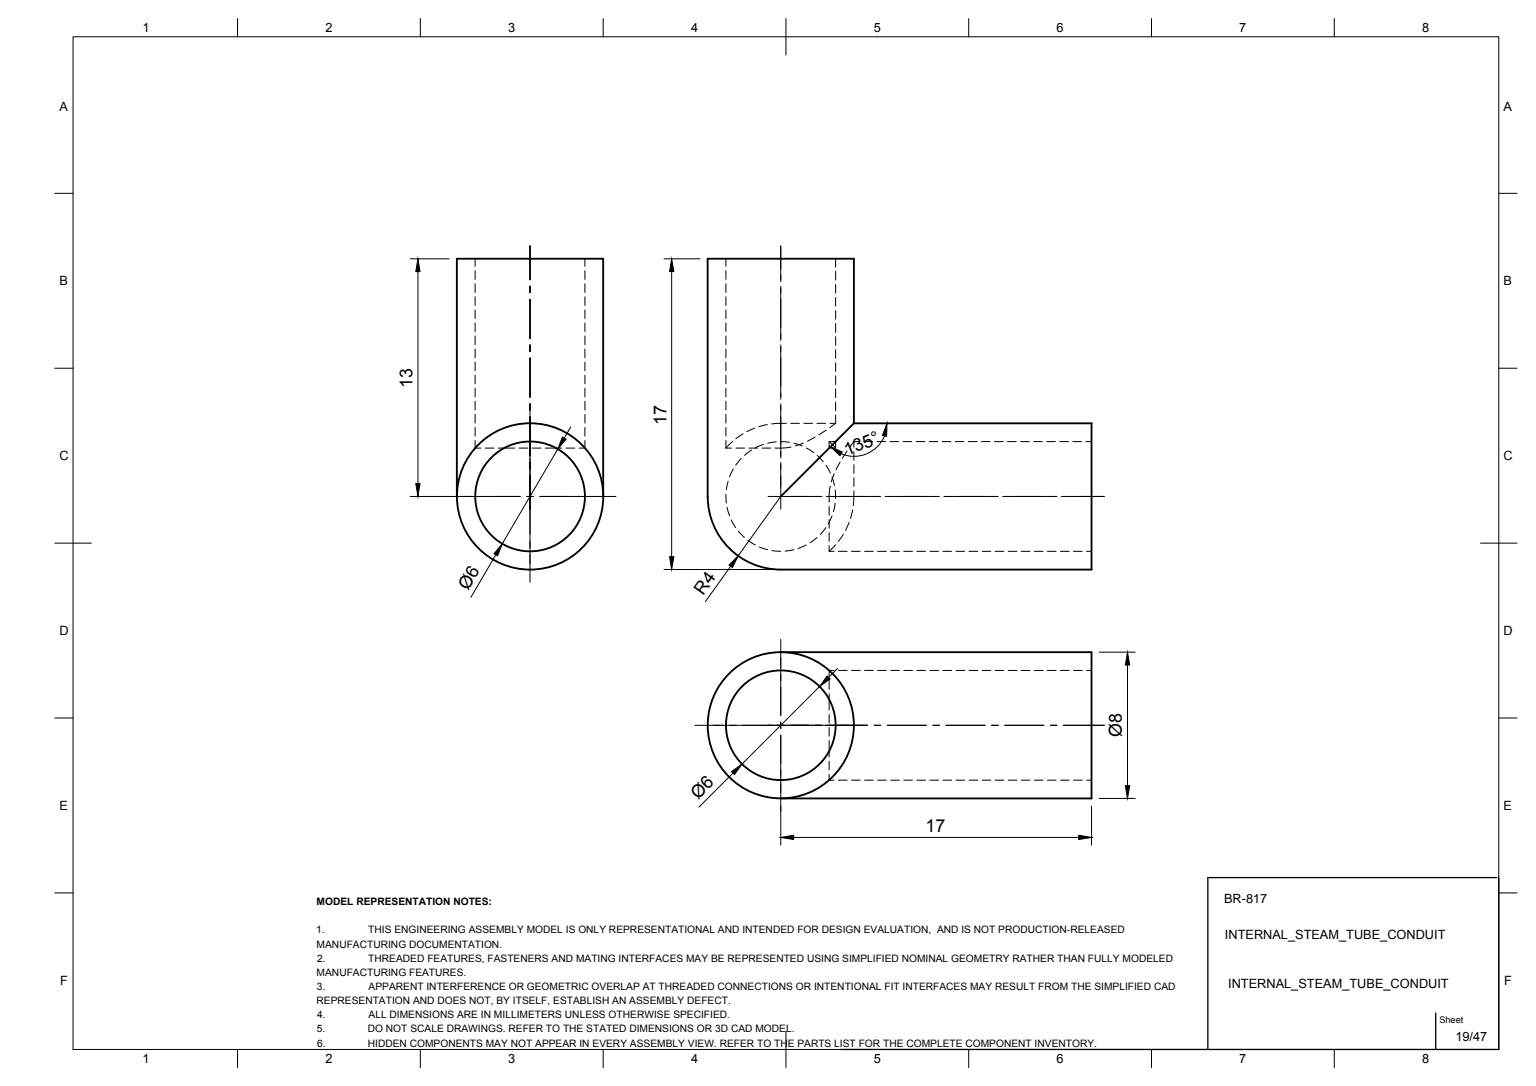
ISO-10303-21;
HEADER;
FILE_DESCRIPTION((''),'2;1');
FILE_NAME('INTERNAL_STEAM_TUBE_CONDUIT.step','2026-10-01T22:07:29-07:00',(''),(''),'','','');
FILE_SCHEMA (('AUTOMOTIVE_DESIGN { 1 0 10303 214 3 1 1 }'));
ENDSEC;
DATA;
#10=MECHANICAL_DESIGN_GEOMETRIC_PRESENTATION_REPRESENTATION('',(#553),#15484);
#11=B_SPLINE_CURVE_WITH_KNOTS('',3,(#13547,#13548,#13549,#13550,#13551,
#13552,#13553,#13554,#13555,#13556,#13557,#13558,#13559,#13560,#13561,#13562,
#13563,#13564,#13565,#13566,#13567,#13568),.UNSPECIFIED.,.F.,.F.,(4,2,2,
2,2,2,2,2,2,2,4),(-0.956775615070491,-0.896341583425282,-0.835907551780074,
-0.715039488489657,-0.596713648012451,-0.478387807535245,-0.36006196705804,
-0.241736126580834,-0.120868063290417,-0.0604340316452086,0.),
 .UNSPECIFIED.) ;
#12=B_SPLINE_CURVE_WITH_KNOTS('',3,(#13586,#13587,#13588,#13589,#13590,
#13591,#13592,#13593,#13594,#13595,#13596,#13597,#13598,#13599,#13600,#13601,
#13602,#13603,#13604,#13605,#13606,#13607),.UNSPECIFIED.,.F.,.F.,(4,2,2,
2,2,2,2,2,2,2,4),(0.,0.0604340316452085,0.120868063290417,0.241736126580834,
0.36006196705804,0.478387807535245,0.596713648012451,0.715039488489657,
0.835907551780074,0.896341583425282,0.956775615070491),.UNSPECIFIED.) ;
#13=ELLIPSE('',#8939,0.424264068711929,0.3) ;
#14=ELLIPSE('',#8947,0.565685424949238,0.4) ;
#189=ORIENTED_CLOSED_SHELL('',*,#8262,.F.) ;
#190=ORIENTED_CLOSED_SHELL('',*,#8263,.F.) ;
#191=BREP_WITH_VOIDS('INTERNAL_STEAM_TUBE_CONDUIT',#8264,(#189,#190)) ;
#193=SPHERICAL_SURFACE('',#8933,0.3) ;
#194=SPHERICAL_SURFACE('',#8935,0.4) ;
#195=SPHERICAL_SURFACE('',#8964,0.4) ;
#196=SPHERICAL_SURFACE('',#8965,0.4) ;
#197=SPHERICAL_SURFACE('',#8966,0.4) ;
#483=SHAPE_REPRESENTATION_RELATIONSHIP('SRR','None',#15632,#518) ;
#518=ADVANCED_BREP_SHAPE_REPRESENTATION('',(#191),#15456) ;
#553=STYLED_ITEM('',(#15836),#191) ;
#667=CYLINDRICAL_SURFACE('',#8938,0.3) ;
#668=CYLINDRICAL_SURFACE('',#8940,0.3) ;
#669=CYLINDRICAL_SURFACE('',#8944,0.4) ;
#670=CYLINDRICAL_SURFACE('',#8946,0.4) ;
#671=CYLINDRICAL_SURFACE('',#8953,0.4) ;
#672=CYLINDRICAL_SURFACE('',#8955,0.4) ;
#673=CYLINDRICAL_SURFACE('',#8958,0.3) ;
#674=CYLINDRICAL_SURFACE('',#8961,0.3) ;
#859=FACE_BOUND('',#2058,.T.) ;
#860=FACE_BOUND('',#2062,.T.) ;
#976=CIRCLE('',#8934,0.3) ;
#977=CIRCLE('',#8936,0.3) ;
#978=CIRCLE('',#8937,0.3) ;
#979=CIRCLE('',#8942,0.4) ;
#980=CIRCLE('',#8943,0.3) ;
#981=CIRCLE('',#8945,0.4) ;
#982=CIRCLE('',#8948,0.4) ;
#983=CIRCLE('',#8949,0.4) ;
#984=CIRCLE('',#8951,0.4) ;
#985=CIRCLE('',#8952,0.3) ;
#986=CIRCLE('',#8954,0.4) ;
#987=CIRCLE('',#8956,0.4) ;
#988=CIRCLE('',#8957,0.4) ;
#989=CIRCLE('',#8959,0.3) ;
#990=CIRCLE('',#8960,0.3) ;
#991=CIRCLE('',#8962,0.3) ;
#992=CIRCLE('',#8963,0.3) ;
#1504=FACE_OUTER_BOUND('',#2053,.T.) ;
#1505=FACE_OUTER_BOUND('',#2054,.T.) ;
#1506=FACE_OUTER_BOUND('',#2055,.T.) ;
#1507=FACE_OUTER_BOUND('',#2056,.T.) ;
#1508=FACE_OUTER_BOUND('',#2057,.T.) ;
#1509=FACE_OUTER_BOUND('',#2059,.T.) ;
#1510=FACE_OUTER_BOUND('',#2060,.T.) ;
#1511=FACE_OUTER_BOUND('',#2061,.T.) ;
#1512=FACE_OUTER_BOUND('',#2063,.T.) ;
#1513=FACE_OUTER_BOUND('',#2064,.T.) ;
#1514=FACE_OUTER_BOUND('',#2065,.T.) ;
#1515=FACE_OUTER_BOUND('',#2066,.T.) ;
#1516=FACE_OUTER_BOUND('',#2067,.T.) ;
#1517=FACE_OUTER_BOUND('',#2068,.T.) ;
#1518=FACE_OUTER_BOUND('',#2069,.T.) ;
#2053=EDGE_LOOP('',(#5851,#5852)) ;
#2054=EDGE_LOOP('',(#5853,#5854)) ;
#2055=EDGE_LOOP('',(#5855,#5856)) ;
#2056=EDGE_LOOP('',(#5857,#5858)) ;
#2057=EDGE_LOOP('',(#5859)) ;
#2058=EDGE_LOOP('',(#5860)) ;
#2059=EDGE_LOOP('',(#5861,#5862)) ;
#2060=EDGE_LOOP('',(#5863,#5864,#5865,#5866,#5867,#5868)) ;
#2061=EDGE_LOOP('',(#5869)) ;
#2062=EDGE_LOOP('',(#5870)) ;
#2063=EDGE_LOOP('',(#5871,#5872)) ;
#2064=EDGE_LOOP('',(#5873,#5874,#5875,#5876,#5877,#5878)) ;
#2065=EDGE_LOOP('',(#5879,#5880,#5881,#5882,#5883,#5884)) ;
#2066=EDGE_LOOP('',(#5885,#5886,#5887,#5888,#5889,#5890)) ;
#2067=EDGE_LOOP('',(#5891,#5892,#5893,#5894)) ;
#2068=EDGE_LOOP('',(#5895,#5896,#5897)) ;
#2069=EDGE_LOOP('',(#5898,#5899,#5900)) ;
#2638=LINE('',#13576,#3112) ;
#2639=LINE('',#13611,#3113) ;
#2640=LINE('',#13617,#3114) ;
#2641=LINE('',#13621,#3115) ;
#3112=VECTOR('',#10657,0.4) ;
#3113=VECTOR('',#10672,0.4) ;
#3114=VECTOR('',#10681,0.3) ;
#3115=VECTOR('',#10686,0.3) ;
#3581=VERTEX_POINT('',#13528) ;
#3582=VERTEX_POINT('',#13529) ;
#3583=VERTEX_POINT('',#13532) ;
#3584=VERTEX_POINT('',#13533) ;
#3585=VERTEX_POINT('',#13540) ;
#3586=VERTEX_POINT('',#13542) ;
#3587=VERTEX_POINT('',#13545) ;
#3588=VERTEX_POINT('',#13546) ;
#3589=VERTEX_POINT('',#13571) ;
#3590=VERTEX_POINT('',#13572) ;
#3591=VERTEX_POINT('',#13574) ;
#3592=VERTEX_POINT('',#13579) ;
#3593=VERTEX_POINT('',#13581) ;
#3594=VERTEX_POINT('',#13584) ;
#3595=VERTEX_POINT('',#13585) ;
#3596=VERTEX_POINT('',#13610) ;
#3597=VERTEX_POINT('',#13615) ;
#3598=VERTEX_POINT('',#13620) ;
#4430=EDGE_CURVE('',#3581,#3582,#976,.T.) ;
#4431=EDGE_CURVE('',#3583,#3584,#977,.T.) ;
#4432=EDGE_CURVE('',#3584,#3583,#978,.T.) ;
#4433=EDGE_CURVE('',#3583,#3584,#13,.T.) ;
#4434=EDGE_CURVE('',#3585,#3585,#979,.T.) ;
#4435=EDGE_CURVE('',#3586,#3586,#980,.T.) ;
#4436=EDGE_CURVE('',#3587,#3588,#11,.T.) ;
#4437=EDGE_CURVE('',#3587,#3588,#981,.T.) ;
#4438=EDGE_CURVE('',#3589,#3590,#14,.T.) ;
#4439=EDGE_CURVE('',#3591,#3590,#982,.T.) ;
#4440=EDGE_CURVE('',#3591,#3585,#2638,.T.) ;
#4441=EDGE_CURVE('',#3589,#3591,#983,.T.) ;
#4442=EDGE_CURVE('',#3592,#3592,#984,.T.) ;
#4443=EDGE_CURVE('',#3593,#3593,#985,.T.) ;
#4444=EDGE_CURVE('',#3594,#3595,#12,.T.) ;
#4445=EDGE_CURVE('',#3595,#3594,#986,.T.) ;
#4446=EDGE_CURVE('',#3592,#3596,#2639,.T.) ;
#4447=EDGE_CURVE('',#3590,#3596,#987,.T.) ;
#4448=EDGE_CURVE('',#3596,#3589,#988,.T.) ;
#4449=EDGE_CURVE('',#3587,#3597,#989,.T.) ;
#4450=EDGE_CURVE('',#3597,#3593,#2640,.T.) ;
#4451=EDGE_CURVE('',#3597,#3588,#990,.T.) ;
#4452=EDGE_CURVE('',#3586,#3598,#2641,.T.) ;
#4453=EDGE_CURVE('',#3598,#3594,#991,.T.) ;
#4454=EDGE_CURVE('',#3595,#3598,#992,.T.) ;
#5851=ORIENTED_EDGE('',*,*,#4430,.T.) ;
#5852=ORIENTED_EDGE('',*,*,#4430,.F.) ;
#5853=ORIENTED_EDGE('',*,*,#4431,.F.) ;
#5854=ORIENTED_EDGE('',*,*,#4432,.F.) ;
#5855=ORIENTED_EDGE('',*,*,#4432,.T.) ;
#5856=ORIENTED_EDGE('',*,*,#4433,.T.) ;
#5857=ORIENTED_EDGE('',*,*,#4431,.T.) ;
#5858=ORIENTED_EDGE('',*,*,#4433,.F.) ;
#5859=ORIENTED_EDGE('',*,*,#4434,.T.) ;
#5860=ORIENTED_EDGE('',*,*,#4435,.T.) ;
#5861=ORIENTED_EDGE('',*,*,#4436,.T.) ;
#5862=ORIENTED_EDGE('',*,*,#4437,.F.) ;
#5863=ORIENTED_EDGE('',*,*,#4438,.T.) ;
#5864=ORIENTED_EDGE('',*,*,#4439,.F.) ;
#5865=ORIENTED_EDGE('',*,*,#4440,.T.) ;
#5866=ORIENTED_EDGE('',*,*,#4434,.F.) ;
#5867=ORIENTED_EDGE('',*,*,#4440,.F.) ;
#5868=ORIENTED_EDGE('',*,*,#4441,.F.) ;
#5869=ORIENTED_EDGE('',*,*,#4442,.T.) ;
#5870=ORIENTED_EDGE('',*,*,#4443,.T.) ;
#5871=ORIENTED_EDGE('',*,*,#4444,.F.) ;
#5872=ORIENTED_EDGE('',*,*,#4445,.F.) ;
#5873=ORIENTED_EDGE('',*,*,#4442,.F.) ;
#5874=ORIENTED_EDGE('',*,*,#4446,.T.) ;
#5875=ORIENTED_EDGE('',*,*,#4447,.F.) ;
#5876=ORIENTED_EDGE('',*,*,#4438,.F.) ;
#5877=ORIENTED_EDGE('',*,*,#4448,.F.) ;
#5878=ORIENTED_EDGE('',*,*,#4446,.F.) ;
#5879=ORIENTED_EDGE('',*,*,#4449,.T.) ;
#5880=ORIENTED_EDGE('',*,*,#4450,.T.) ;
#5881=ORIENTED_EDGE('',*,*,#4443,.F.) ;
#5882=ORIENTED_EDGE('',*,*,#4450,.F.) ;
#5883=ORIENTED_EDGE('',*,*,#4451,.T.) ;
#5884=ORIENTED_EDGE('',*,*,#4436,.F.) ;
#5885=ORIENTED_EDGE('',*,*,#4435,.F.) ;
#5886=ORIENTED_EDGE('',*,*,#4452,.T.) ;
#5887=ORIENTED_EDGE('',*,*,#4453,.T.) ;
#5888=ORIENTED_EDGE('',*,*,#4444,.T.) ;
#5889=ORIENTED_EDGE('',*,*,#4454,.T.) ;
#5890=ORIENTED_EDGE('',*,*,#4452,.F.) ;
#5891=ORIENTED_EDGE('',*,*,#4447,.T.) ;
#5892=ORIENTED_EDGE('',*,*,#4448,.T.) ;
#5893=ORIENTED_EDGE('',*,*,#4441,.T.) ;
#5894=ORIENTED_EDGE('',*,*,#4439,.T.) ;
#5895=ORIENTED_EDGE('',*,*,#4449,.F.) ;
#5896=ORIENTED_EDGE('',*,*,#4437,.T.) ;
#5897=ORIENTED_EDGE('',*,*,#4451,.F.) ;
#5898=ORIENTED_EDGE('',*,*,#4445,.T.) ;
#5899=ORIENTED_EDGE('',*,*,#4453,.F.) ;
#5900=ORIENTED_EDGE('',*,*,#4454,.F.) ;
#7634=PLANE('',#8941) ;
#7635=PLANE('',#8950) ;
#7891=ADVANCED_FACE('',(#1504),#193,.F.) ;
#7892=ADVANCED_FACE('',(#1505),#194,.T.) ;
#7893=ADVANCED_FACE('',(#1506),#667,.F.) ;
#7894=ADVANCED_FACE('',(#1507),#668,.F.) ;
#7895=ADVANCED_FACE('',(#1508,#859),#7634,.T.) ;
#7896=ADVANCED_FACE('',(#1509),#669,.T.) ;
#7897=ADVANCED_FACE('',(#1510),#670,.T.) ;
#7898=ADVANCED_FACE('',(#1511,#860),#7635,.T.) ;
#7899=ADVANCED_FACE('',(#1512),#671,.T.) ;
#7900=ADVANCED_FACE('',(#1513),#672,.T.) ;
#7901=ADVANCED_FACE('',(#1514),#673,.F.) ;
#7902=ADVANCED_FACE('',(#1515),#674,.F.) ;
#7903=ADVANCED_FACE('',(#1516),#195,.T.) ;
#7904=ADVANCED_FACE('',(#1517),#196,.T.) ;
#7905=ADVANCED_FACE('',(#1518),#197,.T.) ;
#8262=CLOSED_SHELL('',(#7891)) ;
#8263=CLOSED_SHELL('',(#7892,#7893,#7894)) ;
#8264=CLOSED_SHELL('',(#7895,#7896,#7897,#7898,#7899,#7900,#7901,#7902,
#7903,#7904,#7905)) ;
#8932=AXIS2_PLACEMENT_3D('',#13526,#10623,#10624) ;
#8933=AXIS2_PLACEMENT_3D('',#13527,#10625,#10626) ;
#8934=AXIS2_PLACEMENT_3D('',#13530,#10627,#10628) ;
#8935=AXIS2_PLACEMENT_3D('',#13531,#10629,#10630) ;
#8936=AXIS2_PLACEMENT_3D('',#13534,#10631,#10632) ;
#8937=AXIS2_PLACEMENT_3D('',#13535,#10633,#10634) ;
#8938=AXIS2_PLACEMENT_3D('',#13536,#10635,#10636) ;
#8939=AXIS2_PLACEMENT_3D('',#13537,#10637,#10638) ;
#8940=AXIS2_PLACEMENT_3D('',#13538,#10639,#10640) ;
#8941=AXIS2_PLACEMENT_3D('',#13539,#10641,#10642) ;
#8942=AXIS2_PLACEMENT_3D('',#13541,#10643,#10644) ;
#8943=AXIS2_PLACEMENT_3D('',#13543,#10645,#10646) ;
#8944=AXIS2_PLACEMENT_3D('',#13544,#10647,#10648) ;
#8945=AXIS2_PLACEMENT_3D('',#13569,#10649,#10650) ;
#8946=AXIS2_PLACEMENT_3D('',#13570,#10651,#10652) ;
#8947=AXIS2_PLACEMENT_3D('',#13573,#10653,#10654) ;
#8948=AXIS2_PLACEMENT_3D('',#13575,#10655,#10656) ;
#8949=AXIS2_PLACEMENT_3D('',#13577,#10658,#10659) ;
#8950=AXIS2_PLACEMENT_3D('',#13578,#10660,#10661) ;
#8951=AXIS2_PLACEMENT_3D('',#13580,#10662,#10663) ;
#8952=AXIS2_PLACEMENT_3D('',#13582,#10664,#10665) ;
#8953=AXIS2_PLACEMENT_3D('',#13583,#10666,#10667) ;
#8954=AXIS2_PLACEMENT_3D('',#13608,#10668,#10669) ;
#8955=AXIS2_PLACEMENT_3D('',#13609,#10670,#10671) ;
#8956=AXIS2_PLACEMENT_3D('',#13612,#10673,#10674) ;
#8957=AXIS2_PLACEMENT_3D('',#13613,#10675,#10676) ;
#8958=AXIS2_PLACEMENT_3D('',#13614,#10677,#10678) ;
#8959=AXIS2_PLACEMENT_3D('',#13616,#10679,#10680) ;
#8960=AXIS2_PLACEMENT_3D('',#13618,#10682,#10683) ;
#8961=AXIS2_PLACEMENT_3D('',#13619,#10684,#10685) ;
#8962=AXIS2_PLACEMENT_3D('',#13622,#10687,#10688) ;
#8963=AXIS2_PLACEMENT_3D('',#13623,#10689,#10690) ;
#8964=AXIS2_PLACEMENT_3D('',#13624,#10691,#10692) ;
#8965=AXIS2_PLACEMENT_3D('',#13625,#10693,#10694) ;
#8966=AXIS2_PLACEMENT_3D('',#13626,#10695,#10696) ;
#10623=DIRECTION('axis',(0.,0.,1.)) ;
#10624=DIRECTION('refdir',(1.,0.,0.)) ;
#10625=DIRECTION('center_axis',(0.,0.,1.)) ;
#10626=DIRECTION('ref_axis',(1.,0.,0.)) ;
#10627=DIRECTION('center_axis',(0.,1.,0.)) ;
#10628=DIRECTION('ref_axis',(-1.,0.,0.)) ;
#10629=DIRECTION('center_axis',(0.,0.,1.)) ;
#10630=DIRECTION('ref_axis',(1.,0.,0.)) ;
#10631=DIRECTION('center_axis',(-1.,0.,0.)) ;
#10632=DIRECTION('ref_axis',(0.,0.,-1.)) ;
#10633=DIRECTION('center_axis',(0.,0.,1.)) ;
#10634=DIRECTION('ref_axis',(1.,0.,0.)) ;
#10635=DIRECTION('center_axis',(0.,0.,1.)) ;
#10636=DIRECTION('ref_axis',(1.,0.,0.)) ;
#10637=DIRECTION('center_axis',(-0.707106781186548,0.,-0.707106781186548)) ;
#10638=DIRECTION('ref_axis',(0.707106781186548,0.,-0.707106781186548)) ;
#10639=DIRECTION('center_axis',(1.,0.,0.)) ;
#10640=DIRECTION('ref_axis',(0.,0.,-1.)) ;
#10641=DIRECTION('center_axis',(0.,0.,-1.)) ;
#10642=DIRECTION('ref_axis',(-1.,0.,0.)) ;
#10643=DIRECTION('center_axis',(0.,0.,-1.)) ;
#10644=DIRECTION('ref_axis',(1.,0.,0.)) ;
#10645=DIRECTION('center_axis',(0.,0.,1.)) ;
#10646=DIRECTION('ref_axis',(1.,0.,0.)) ;
#10647=DIRECTION('center_axis',(0.,0.,1.)) ;
#10648=DIRECTION('ref_axis',(1.,0.,0.)) ;
#10649=DIRECTION('center_axis',(0.,0.,1.)) ;
#10650=DIRECTION('ref_axis',(1.,0.,0.)) ;
#10651=DIRECTION('center_axis',(0.,0.,1.)) ;
#10652=DIRECTION('ref_axis',(1.,0.,0.)) ;
#10653=DIRECTION('center_axis',(-0.707106781186548,0.,-0.707106781186548)) ;
#10654=DIRECTION('ref_axis',(0.707106781186547,0.,-0.707106781186547)) ;
#10655=DIRECTION('center_axis',(0.,0.,1.)) ;
#10656=DIRECTION('ref_axis',(1.,0.,0.)) ;
#10657=DIRECTION('',(0.,0.,-1.)) ;
#10658=DIRECTION('center_axis',(0.,0.,1.)) ;
#10659=DIRECTION('ref_axis',(1.,0.,0.)) ;
#10660=DIRECTION('center_axis',(1.,0.,0.)) ;
#10661=DIRECTION('ref_axis',(0.,0.,-1.)) ;
#10662=DIRECTION('center_axis',(1.,0.,0.)) ;
#10663=DIRECTION('ref_axis',(0.,0.,-1.)) ;
#10664=DIRECTION('center_axis',(-1.,0.,0.)) ;
#10665=DIRECTION('ref_axis',(0.,0.,-1.)) ;
#10666=DIRECTION('center_axis',(1.,0.,0.)) ;
#10667=DIRECTION('ref_axis',(0.,0.,-1.)) ;
#10668=DIRECTION('center_axis',(-1.,0.,0.)) ;
#10669=DIRECTION('ref_axis',(0.,0.,-1.)) ;
#10670=DIRECTION('center_axis',(1.,0.,0.)) ;
#10671=DIRECTION('ref_axis',(0.,0.,-1.)) ;
#10672=DIRECTION('',(-1.,0.,0.)) ;
#10673=DIRECTION('center_axis',(-1.,0.,0.)) ;
#10674=DIRECTION('ref_axis',(0.,0.,-1.)) ;
#10675=DIRECTION('center_axis',(-1.,0.,0.)) ;
#10676=DIRECTION('ref_axis',(0.,0.,-1.)) ;
#10677=DIRECTION('center_axis',(1.,0.,0.)) ;
#10678=DIRECTION('ref_axis',(0.,0.,-1.)) ;
#10679=DIRECTION('center_axis',(-1.,0.,0.)) ;
#10680=DIRECTION('ref_axis',(0.,0.,-1.)) ;
#10681=DIRECTION('',(1.,0.,0.)) ;
#10682=DIRECTION('center_axis',(-1.,0.,0.)) ;
#10683=DIRECTION('ref_axis',(0.,0.,-1.)) ;
#10684=DIRECTION('center_axis',(0.,0.,1.)) ;
#10685=DIRECTION('ref_axis',(1.,0.,0.)) ;
#10686=DIRECTION('',(0.,0.,1.)) ;
#10687=DIRECTION('center_axis',(0.,0.,1.)) ;
#10688=DIRECTION('ref_axis',(1.,0.,0.)) ;
#10689=DIRECTION('center_axis',(0.,0.,1.)) ;
#10690=DIRECTION('ref_axis',(1.,0.,0.)) ;
#10691=DIRECTION('center_axis',(0.577350269189626,0.577350269189626,0.577350269189626)) ;
#10692=DIRECTION('ref_axis',(-0.707106781186548,0.,0.707106781186548)) ;
#10693=DIRECTION('center_axis',(0.,0.,1.)) ;
#10694=DIRECTION('ref_axis',(1.,0.,0.)) ;
#10695=DIRECTION('center_axis',(1.,0.,0.)) ;
#10696=DIRECTION('ref_axis',(0.,-1.,0.)) ;
#13526=CARTESIAN_POINT('',(0.,0.,0.)) ;
#13527=CARTESIAN_POINT('Origin',(2.5,1.4,3.4)) ;
#13528=CARTESIAN_POINT('',(2.5,1.4,3.1)) ;
#13529=CARTESIAN_POINT('',(2.5,1.4,3.7)) ;
#13530=CARTESIAN_POINT('Origin',(2.5,1.4,3.4)) ;
#13531=CARTESIAN_POINT('Origin',(2.5,1.4,3.4)) ;
#13532=CARTESIAN_POINT('',(2.76457513110646,1.54142135623731,3.13542486889354)) ;
#13533=CARTESIAN_POINT('',(2.76457513110646,1.25857864376269,3.13542486889354)) ;
#13534=CARTESIAN_POINT('Origin',(2.76457513110646,1.4,3.4)) ;
#13535=CARTESIAN_POINT('Origin',(2.5,1.4,3.13542486889354)) ;
#13536=CARTESIAN_POINT('Origin',(2.5,1.4,2.55)) ;
#13537=CARTESIAN_POINT('Origin',(2.5,1.4,3.4)) ;
#13538=CARTESIAN_POINT('Origin',(3.15,1.4,3.4)) ;
#13539=CARTESIAN_POINT('Origin',(2.5,1.4,1.7)) ;
#13540=CARTESIAN_POINT('',(2.1,1.4,1.7)) ;
#13541=CARTESIAN_POINT('Origin',(2.5,1.4,1.7)) ;
#13542=CARTESIAN_POINT('',(2.2,1.4,1.7)) ;
#13543=CARTESIAN_POINT('Origin',(2.5,1.4,1.7)) ;
#13544=CARTESIAN_POINT('Origin',(2.5,1.4,2.55)) ;
#13545=CARTESIAN_POINT('',(2.76457513110646,1.1,3.4)) ;
#13546=CARTESIAN_POINT('',(2.76457513110646,1.7,3.4)) ;
#13547=CARTESIAN_POINT('Ctrl Pts',(2.76457513110646,1.1,3.4)) ;
#13548=CARTESIAN_POINT('Ctrl Pts',(2.76457513110646,1.1,3.37985532278493)) ;
#13549=CARTESIAN_POINT('Ctrl Pts',(2.76694665658319,1.1020492278835,3.3596364158444)) ;
#13550=CARTESIAN_POINT('Ctrl Pts',(2.7756634705603,1.11009513514317,3.32025634008317)) ;
#13551=CARTESIAN_POINT('Ctrl Pts',(2.78197027038471,1.11608711674642,3.30108570205275)) ;
#13552=CARTESIAN_POINT('Ctrl Pts',(2.80406356980255,1.1392312552828,3.24650091982942)) ;
#13553=CARTESIAN_POINT('Ctrl Pts',(2.82281865282694,1.16181405724795,3.21392187404012)) ;
#13554=CARTESIAN_POINT('Ctrl Pts',(2.85507155223138,1.21337388114196,3.16236205014611)) ;
#13555=CARTESIAN_POINT('Ctrl Pts',(2.87117243484146,1.24601764444721,3.13945139911714)) ;
#13556=CARTESIAN_POINT('Ctrl Pts',(2.89371396047987,1.31957074694018,3.10823419970573)) ;
#13557=CARTESIAN_POINT('Ctrl Pts',(2.9,1.36055805317426,3.1)) ;
#13558=CARTESIAN_POINT('Ctrl Pts',(2.9,1.43944194682574,3.1)) ;
#13559=CARTESIAN_POINT('Ctrl Pts',(2.89371396047987,1.48042925305982,3.10823419970573)) ;
#13560=CARTESIAN_POINT('Ctrl Pts',(2.87117243484146,1.55398235555279,3.13945139911714)) ;
#13561=CARTESIAN_POINT('Ctrl Pts',(2.85507155223138,1.58662611885804,3.16236205014611)) ;
#13562=CARTESIAN_POINT('Ctrl Pts',(2.82281865282694,1.63818594275205,3.21392187404012)) ;
#13563=CARTESIAN_POINT('Ctrl Pts',(2.80406356980255,1.6607687447172,3.24650091982942)) ;
#13564=CARTESIAN_POINT('Ctrl Pts',(2.78197027038471,1.68391288325358,3.30108570205275)) ;
#13565=CARTESIAN_POINT('Ctrl Pts',(2.7756634705603,1.68990486485683,3.32025634008317)) ;
#13566=CARTESIAN_POINT('Ctrl Pts',(2.76694665658319,1.6979507721165,3.3596364158444)) ;
#13567=CARTESIAN_POINT('Ctrl Pts',(2.76457513110646,1.7,3.37985532278493)) ;
#13568=CARTESIAN_POINT('Ctrl Pts',(2.76457513110646,1.7,3.4)) ;
#13569=CARTESIAN_POINT('Origin',(2.5,1.4,3.4)) ;
#13570=CARTESIAN_POINT('Origin',(2.5,1.4,2.55)) ;
#13571=CARTESIAN_POINT('',(2.5,1.8,3.4)) ;
#13572=CARTESIAN_POINT('',(2.5,1.,3.4)) ;
#13573=CARTESIAN_POINT('Origin',(2.5,1.4,3.4)) ;
#13574=CARTESIAN_POINT('',(2.1,1.4,3.4)) ;
#13575=CARTESIAN_POINT('Origin',(2.5,1.4,3.4)) ;
#13576=CARTESIAN_POINT('',(2.1,1.4,2.55)) ;
#13577=CARTESIAN_POINT('Origin',(2.5,1.4,3.4)) ;
#13578=CARTESIAN_POINT('Origin',(3.8,1.4,3.4)) ;
#13579=CARTESIAN_POINT('',(3.8,1.4,3.8)) ;
#13580=CARTESIAN_POINT('Origin',(3.8,1.4,3.4)) ;
#13581=CARTESIAN_POINT('',(3.8,1.4,3.7)) ;
#13582=CARTESIAN_POINT('Origin',(3.8,1.4,3.4)) ;
#13583=CARTESIAN_POINT('Origin',(3.15,1.4,3.4)) ;
#13584=CARTESIAN_POINT('',(2.5,1.1,3.13542486889354)) ;
#13585=CARTESIAN_POINT('',(2.5,1.7,3.13542486889354)) ;
#13586=CARTESIAN_POINT('Ctrl Pts',(2.5,1.1,3.13542486889354)) ;
#13587=CARTESIAN_POINT('Ctrl Pts',(2.52014467721507,1.1,3.13542486889354)) ;
#13588=CARTESIAN_POINT('Ctrl Pts',(2.5403635841556,1.1020492278835,3.13305334341681)) ;
#13589=CARTESIAN_POINT('Ctrl Pts',(2.57974365991683,1.11009513514317,3.1243365294397)) ;
#13590=CARTESIAN_POINT('Ctrl Pts',(2.59891429794725,1.11608711674642,3.11802972961529)) ;
#13591=CARTESIAN_POINT('Ctrl Pts',(2.65349908017058,1.1392312552828,3.09593643019745)) ;
#13592=CARTESIAN_POINT('Ctrl Pts',(2.68607812595988,1.16181405724795,3.07718134717306)) ;
#13593=CARTESIAN_POINT('Ctrl Pts',(2.73763794985389,1.21337388114196,3.04492844776862)) ;
#13594=CARTESIAN_POINT('Ctrl Pts',(2.76054860088286,1.24601764444721,3.02882756515854)) ;
#13595=CARTESIAN_POINT('Ctrl Pts',(2.79176580029427,1.31957074694018,3.00628603952013)) ;
#13596=CARTESIAN_POINT('Ctrl Pts',(2.8,1.36055805317426,3.)) ;
#13597=CARTESIAN_POINT('Ctrl Pts',(2.8,1.43944194682574,3.)) ;
#13598=CARTESIAN_POINT('Ctrl Pts',(2.79176580029427,1.48042925305982,3.00628603952013)) ;
#13599=CARTESIAN_POINT('Ctrl Pts',(2.76054860088286,1.55398235555279,3.02882756515854)) ;
#13600=CARTESIAN_POINT('Ctrl Pts',(2.73763794985389,1.58662611885804,3.04492844776862)) ;
#13601=CARTESIAN_POINT('Ctrl Pts',(2.68607812595988,1.63818594275205,3.07718134717306)) ;
#13602=CARTESIAN_POINT('Ctrl Pts',(2.65349908017058,1.6607687447172,3.09593643019745)) ;
#13603=CARTESIAN_POINT('Ctrl Pts',(2.59891429794725,1.68391288325358,3.11802972961529)) ;
#13604=CARTESIAN_POINT('Ctrl Pts',(2.57974365991683,1.68990486485683,3.1243365294397)) ;
#13605=CARTESIAN_POINT('Ctrl Pts',(2.5403635841556,1.6979507721165,3.13305334341681)) ;
#13606=CARTESIAN_POINT('Ctrl Pts',(2.52014467721507,1.7,3.13542486889354)) ;
#13607=CARTESIAN_POINT('Ctrl Pts',(2.5,1.7,3.13542486889354)) ;
#13608=CARTESIAN_POINT('Origin',(2.5,1.4,3.4)) ;
#13609=CARTESIAN_POINT('Origin',(3.15,1.4,3.4)) ;
#13610=CARTESIAN_POINT('',(2.5,1.4,3.8)) ;
#13611=CARTESIAN_POINT('',(3.15,1.4,3.8)) ;
#13612=CARTESIAN_POINT('Origin',(2.5,1.4,3.4)) ;
#13613=CARTESIAN_POINT('Origin',(2.5,1.4,3.4)) ;
#13614=CARTESIAN_POINT('Origin',(3.15,1.4,3.4)) ;
#13615=CARTESIAN_POINT('',(2.76457513110646,1.4,3.7)) ;
#13616=CARTESIAN_POINT('Origin',(2.76457513110646,1.4,3.4)) ;
#13617=CARTESIAN_POINT('',(3.15,1.4,3.7)) ;
#13618=CARTESIAN_POINT('Origin',(2.76457513110646,1.4,3.4)) ;
#13619=CARTESIAN_POINT('Origin',(2.5,1.4,2.55)) ;
#13620=CARTESIAN_POINT('',(2.2,1.4,3.13542486889354)) ;
#13621=CARTESIAN_POINT('',(2.2,1.4,2.55)) ;
#13622=CARTESIAN_POINT('Origin',(2.5,1.4,3.13542486889354)) ;
#13623=CARTESIAN_POINT('Origin',(2.5,1.4,3.13542486889354)) ;
#13624=CARTESIAN_POINT('Origin',(2.5,1.4,3.4)) ;
#13625=CARTESIAN_POINT('Origin',(2.5,1.4,3.4)) ;
#13626=CARTESIAN_POINT('Origin',(2.5,1.4,3.4)) ;
#15413=UNCERTAINTY_MEASURE_WITH_UNIT(LENGTH_MEASURE(0.001),#15485,
'DISTANCE_ACCURACY_VALUE',
'Maximum model space distance between geometric entities at asserted c
onnectivities') ;
#15441=UNCERTAINTY_MEASURE_WITH_UNIT(LENGTH_MEASURE(0.001),#15485,
'DISTANCE_ACCURACY_VALUE',
'Maximum model space distance between geometric entities at asserted c
onnectivities') ;
#15456=(
GEOMETRIC_REPRESENTATION_CONTEXT(3)
GLOBAL_UNCERTAINTY_ASSIGNED_CONTEXT((#15413))
GLOBAL_UNIT_ASSIGNED_CONTEXT((#15485,#15487,#15488))
REPRESENTATION_CONTEXT('','3D')
) ;
#15484=(
GEOMETRIC_REPRESENTATION_CONTEXT(3)
GLOBAL_UNCERTAINTY_ASSIGNED_CONTEXT((#15441))
GLOBAL_UNIT_ASSIGNED_CONTEXT((#15485,#15487,#15488))
REPRESENTATION_CONTEXT('','3D')
) ;
#15485=(
LENGTH_UNIT()
NAMED_UNIT(*)
SI_UNIT(.CENTI.,.METRE.)
) ;
#15487=(
NAMED_UNIT(*)
PLANE_ANGLE_UNIT()
SI_UNIT($,.RADIAN.)
) ;
#15488=(
NAMED_UNIT(*)
SI_UNIT($,.STERADIAN.)
SOLID_ANGLE_UNIT()
) ;
#15503=SHAPE_DEFINITION_REPRESENTATION(#15551,#15632) ;
#15551=PRODUCT_DEFINITION_SHAPE('',$,#15675) ;
#15632=SHAPE_REPRESENTATION('',(#8932),#15456) ;
#15660=PRODUCT_DEFINITION_CONTEXT('part definition',#15788,'design') ;
#15675=PRODUCT_DEFINITION('INTERNAL_STEAM_TUBE_CONDUIT',
'INTERNAL_STEAM_TUBE_CONDUIT',#15717,#15660) ;
#15717=PRODUCT_DEFINITION_FORMATION('',$,#15804) ;
#15788=APPLICATION_CONTEXT(
'Core Data for Automotive Mechanical Design Process') ;
#15789=PRODUCT_CONTEXT('part definition',#15788,'mechanical') ;
#15804=PRODUCT('INTERNAL_STEAM_TUBE_CONDUIT','INTERNAL_STEAM_TUBE_CONDUIT',
$,(#15789)) ;
#15836=PRESENTATION_STYLE_ASSIGNMENT((#15848)) ;
#15848=SURFACE_STYLE_USAGE(.BOTH.,#15860) ;
#15860=SURFACE_SIDE_STYLE('',(#15872)) ;
#15872=SURFACE_STYLE_FILL_AREA(#15884) ;
#15884=FILL_AREA_STYLE('Surface - Matte',(#15896)) ;
#15896=FILL_AREA_STYLE_COLOUR('Surface - Matte',#15908) ;
#15908=COLOUR_RGB('Surface - Matte', 0.08235294, 0.09019608, 0.10196078) ;
ENDSEC;
END-ISO-10303-21;
